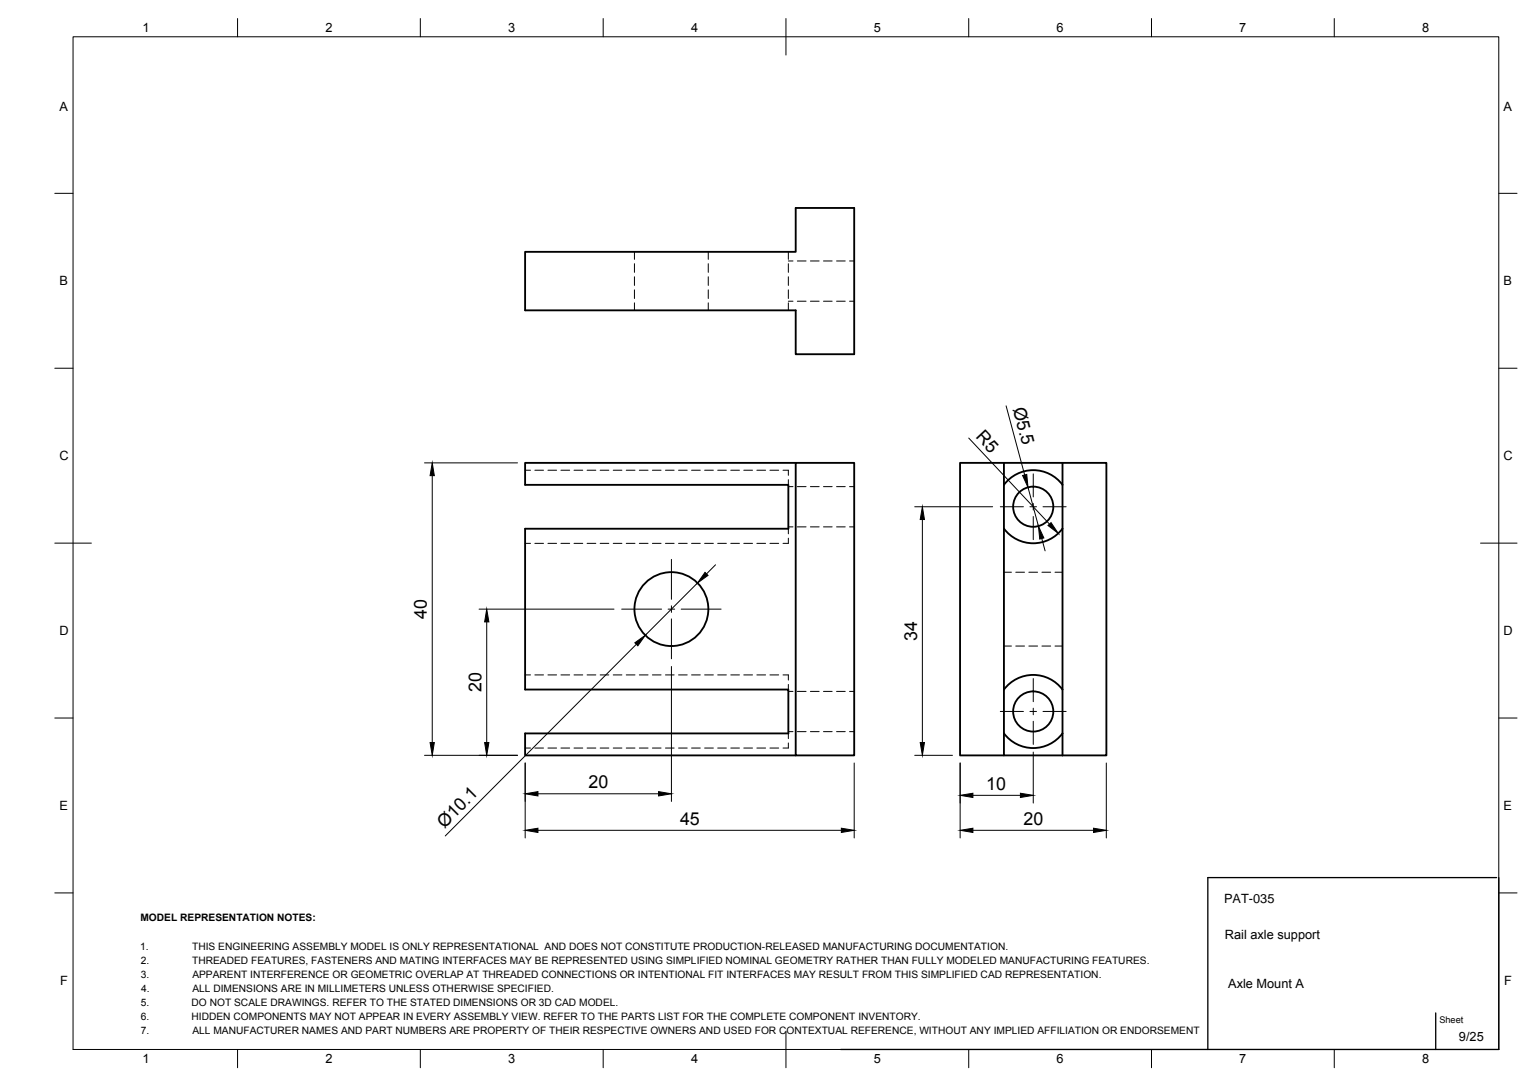
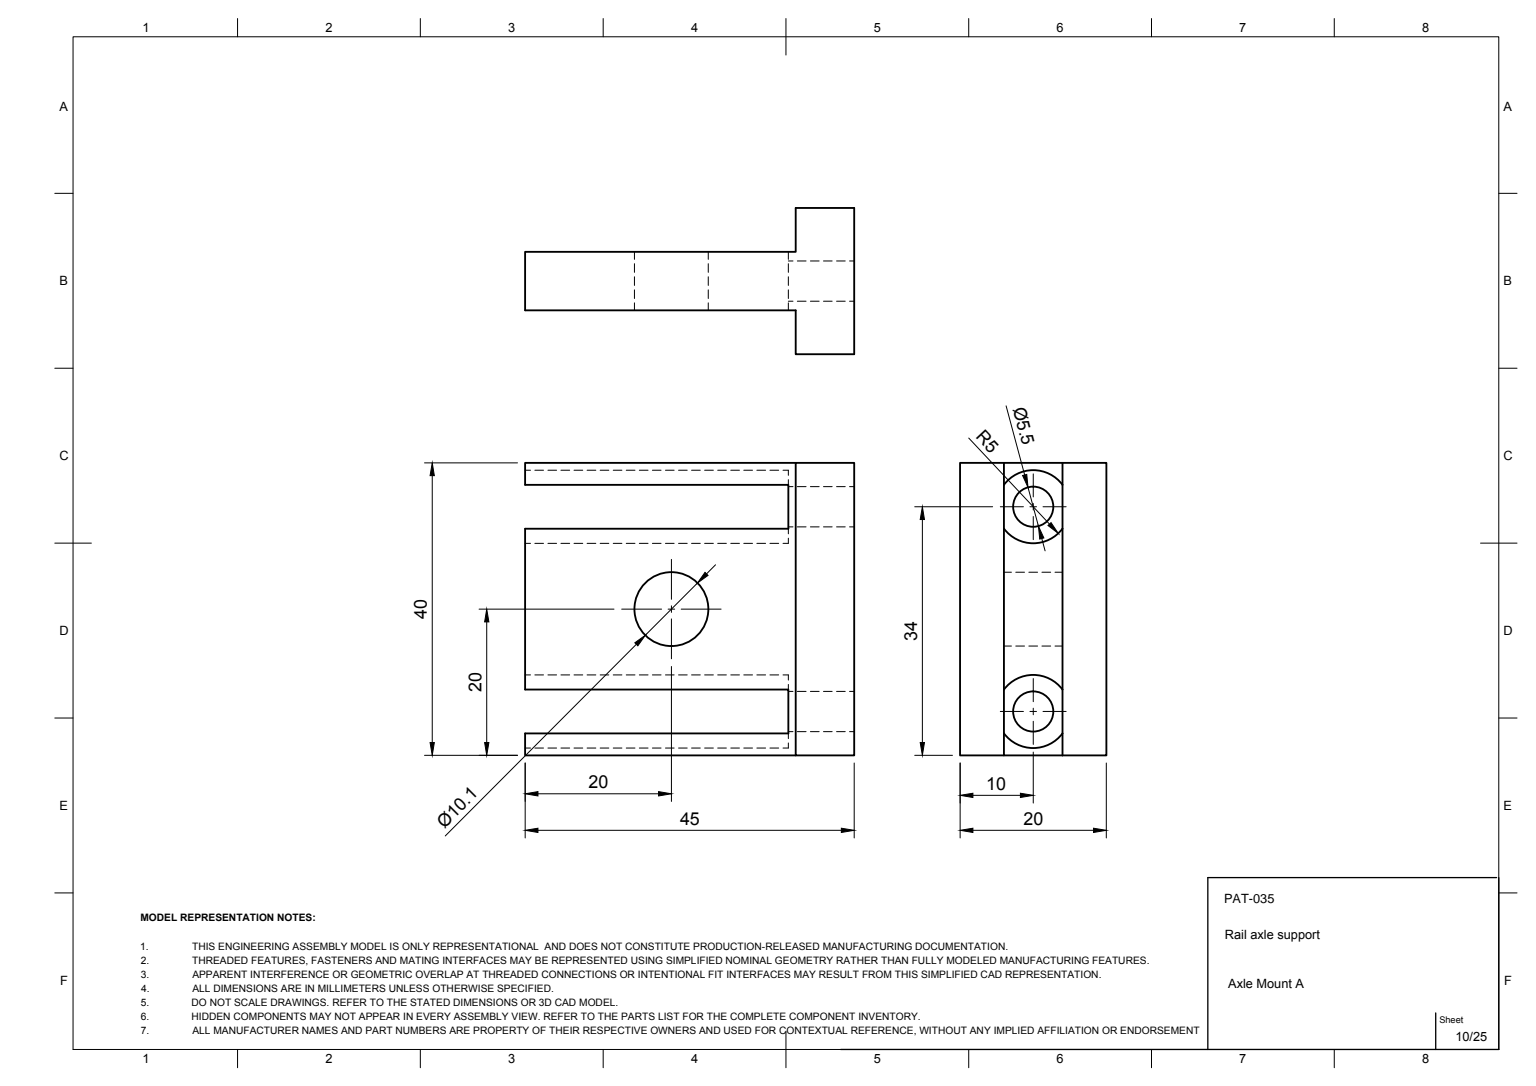
ISO-10303-21;
HEADER;
/* Generated by software containing ST-Developer
 * from STEP Tools, Inc. (www.steptools.com) 
 */

FILE_DESCRIPTION(
/* description */ ('Five-roller gravity conveyor'),
/* implementation_level */ '2;1');

FILE_NAME(
/* name */ 'Axle Mount A.step',
/* time_stamp */ '2026-10-29T15:36:43-07:00',
/* author */ (''),
/* organization */ (''),
/* preprocessor_version */ 'ST-DEVELOPER v20.2',
/* originating_system */ 'Autodesk Translation Framework v15.17.0.0',
/* authorisation */ '');

FILE_SCHEMA (('AUTOMOTIVE_DESIGN { 1 0 10303 214 3 1 1 }'));
ENDSEC;

DATA;
#10=MECHANICAL_DESIGN_GEOMETRIC_PRESENTATION_REPRESENTATION('',(#314),#7806);
#278=SHAPE_REPRESENTATION_RELATIONSHIP('SRR','None',#7915,#296);
#296=ADVANCED_BREP_SHAPE_REPRESENTATION('',(#340),#7788);
#314=STYLED_ITEM('',(#8091),#340);
#340=MANIFOLD_SOLID_BREP('Body1',#4201);
#368=FACE_BOUND('',#951,.T.);
#369=FACE_BOUND('',#955,.T.);
#370=FACE_BOUND('',#957,.T.);
#371=FACE_BOUND('',#969,.T.);
#372=FACE_BOUND('',#973,.T.);
#373=FACE_BOUND('',#974,.T.);
#433=CIRCLE('',#4503,0.5);
#434=CIRCLE('',#4504,0.5);
#435=CIRCLE('',#4506,0.5);
#436=CIRCLE('',#4507,0.5);
#437=CIRCLE('',#4509,0.275);
#438=CIRCLE('',#4511,0.5);
#439=CIRCLE('',#4512,0.5);
#440=CIRCLE('',#4514,0.5);
#441=CIRCLE('',#4515,0.5);
#442=CIRCLE('',#4517,0.275);
#443=CIRCLE('',#4519,0.505);
#444=CIRCLE('',#4524,0.275);
#445=CIRCLE('',#4526,0.275);
#446=CIRCLE('',#4528,0.505);
#600=CYLINDRICAL_SURFACE('',#4502,0.5);
#601=CYLINDRICAL_SURFACE('',#4505,0.5);
#602=CYLINDRICAL_SURFACE('',#4510,0.5);
#603=CYLINDRICAL_SURFACE('',#4513,0.5);
#604=CYLINDRICAL_SURFACE('',#4523,0.275);
#605=CYLINDRICAL_SURFACE('',#4525,0.275);
#606=CYLINDRICAL_SURFACE('',#4527,0.505);
#710=FACE_OUTER_BOUND('',#948,.T.);
#711=FACE_OUTER_BOUND('',#949,.T.);
#712=FACE_OUTER_BOUND('',#950,.T.);
#713=FACE_OUTER_BOUND('',#952,.T.);
#714=FACE_OUTER_BOUND('',#953,.T.);
#715=FACE_OUTER_BOUND('',#954,.T.);
#716=FACE_OUTER_BOUND('',#956,.T.);
#717=FACE_OUTER_BOUND('',#958,.T.);
#718=FACE_OUTER_BOUND('',#959,.T.);
#719=FACE_OUTER_BOUND('',#960,.T.);
#720=FACE_OUTER_BOUND('',#961,.T.);
#721=FACE_OUTER_BOUND('',#962,.T.);
#722=FACE_OUTER_BOUND('',#963,.T.);
#723=FACE_OUTER_BOUND('',#964,.T.);
#724=FACE_OUTER_BOUND('',#965,.T.);
#725=FACE_OUTER_BOUND('',#966,.T.);
#726=FACE_OUTER_BOUND('',#967,.T.);
#727=FACE_OUTER_BOUND('',#968,.T.);
#728=FACE_OUTER_BOUND('',#970,.T.);
#729=FACE_OUTER_BOUND('',#971,.T.);
#730=FACE_OUTER_BOUND('',#972,.T.);
#948=EDGE_LOOP('',(#3054,#3055,#3056,#3057));
#949=EDGE_LOOP('',(#3058,#3059,#3060,#3061));
#950=EDGE_LOOP('',(#3062,#3063,#3064,#3065));
#951=EDGE_LOOP('',(#3066));
#952=EDGE_LOOP('',(#3067,#3068,#3069,#3070));
#953=EDGE_LOOP('',(#3071,#3072,#3073,#3074));
#954=EDGE_LOOP('',(#3075,#3076,#3077,#3078));
#955=EDGE_LOOP('',(#3079));
#956=EDGE_LOOP('',(#3080,#3081,#3082,#3083,#3084,#3085,#3086,#3087,#3088,
#3089,#3090,#3091));
#957=EDGE_LOOP('',(#3092));
#958=EDGE_LOOP('',(#3093,#3094,#3095,#3096));
#959=EDGE_LOOP('',(#3097,#3098,#3099,#3100));
#960=EDGE_LOOP('',(#3101,#3102,#3103,#3104));
#961=EDGE_LOOP('',(#3105,#3106,#3107,#3108));
#962=EDGE_LOOP('',(#3109,#3110,#3111,#3112));
#963=EDGE_LOOP('',(#3113,#3114,#3115,#3116));
#964=EDGE_LOOP('',(#3117,#3118,#3119,#3120));
#965=EDGE_LOOP('',(#3121,#3122,#3123,#3124));
#966=EDGE_LOOP('',(#3125,#3126,#3127,#3128));
#967=EDGE_LOOP('',(#3129,#3130,#3131,#3132));
#968=EDGE_LOOP('',(#3133,#3134,#3135,#3136,#3137,#3138,#3139,#3140,#3141,
#3142,#3143,#3144));
#969=EDGE_LOOP('',(#3145));
#970=EDGE_LOOP('',(#3146,#3147,#3148,#3149,#3150,#3151,#3152,#3153));
#971=EDGE_LOOP('',(#3154,#3155,#3156,#3157,#3158,#3159,#3160,#3161));
#972=EDGE_LOOP('',(#3162,#3163,#3164,#3165));
#973=EDGE_LOOP('',(#3166));
#974=EDGE_LOOP('',(#3167));
#1313=LINE('',#6533,#1654);
#1314=LINE('',#6537,#1655);
#1315=LINE('',#6542,#1656);
#1316=LINE('',#6546,#1657);
#1317=LINE('',#6549,#1658);
#1318=LINE('',#6550,#1659);
#1319=LINE('',#6556,#1660);
#1320=LINE('',#6560,#1661);
#1321=LINE('',#6565,#1662);
#1322=LINE('',#6569,#1663);
#1323=LINE('',#6572,#1664);
#1324=LINE('',#6573,#1665);
#1325=LINE('',#6578,#1666);
#1326=LINE('',#6580,#1667);
#1327=LINE('',#6582,#1668);
#1328=LINE('',#6584,#1669);
#1329=LINE('',#6585,#1670);
#1330=LINE('',#6586,#1671);
#1331=LINE('',#6591,#1672);
#1332=LINE('',#6592,#1673);
#1333=LINE('',#6595,#1674);
#1334=LINE('',#6596,#1675);
#1335=LINE('',#6598,#1676);
#1336=LINE('',#6602,#1677);
#1337=LINE('',#6606,#1678);
#1338=LINE('',#6609,#1679);
#1339=LINE('',#6613,#1680);
#1340=LINE('',#6615,#1681);
#1341=LINE('',#6616,#1682);
#1342=LINE('',#6620,#1683);
#1343=LINE('',#6622,#1684);
#1344=LINE('',#6624,#1685);
#1345=LINE('',#6625,#1686);
#1346=LINE('',#6628,#1687);
#1347=LINE('',#6630,#1688);
#1348=LINE('',#6631,#1689);
#1349=LINE('',#6634,#1690);
#1350=LINE('',#6636,#1691);
#1351=LINE('',#6637,#1692);
#1352=LINE('',#6639,#1693);
#1353=LINE('',#6640,#1694);
#1354=LINE('',#6642,#1695);
#1355=LINE('',#6644,#1696);
#1654=VECTOR('',#5201,1.);
#1655=VECTOR('',#5204,1.);
#1656=VECTOR('',#5209,1.);
#1657=VECTOR('',#5212,1.);
#1658=VECTOR('',#5217,1.);
#1659=VECTOR('',#5218,1.);
#1660=VECTOR('',#5223,1.);
#1661=VECTOR('',#5226,1.);
#1662=VECTOR('',#5231,1.);
#1663=VECTOR('',#5234,1.);
#1664=VECTOR('',#5239,1.);
#1665=VECTOR('',#5240,1.);
#1666=VECTOR('',#5245,1.);
#1667=VECTOR('',#5246,1.);
#1668=VECTOR('',#5247,1.);
#1669=VECTOR('',#5248,1.);
#1670=VECTOR('',#5249,1.);
#1671=VECTOR('',#5250,1.);
#1672=VECTOR('',#5255,1.);
#1673=VECTOR('',#5256,1.);
#1674=VECTOR('',#5259,1.);
#1675=VECTOR('',#5260,1.);
#1676=VECTOR('',#5263,1.);
#1677=VECTOR('',#5268,0.275);
#1678=VECTOR('',#5273,0.275);
#1679=VECTOR('',#5276,0.505);
#1680=VECTOR('',#5281,1.);
#1681=VECTOR('',#5282,1.);
#1682=VECTOR('',#5283,1.);
#1683=VECTOR('',#5286,1.);
#1684=VECTOR('',#5287,1.);
#1685=VECTOR('',#5288,1.);
#1686=VECTOR('',#5289,1.);
#1687=VECTOR('',#5292,1.);
#1688=VECTOR('',#5293,1.);
#1689=VECTOR('',#5294,1.);
#1690=VECTOR('',#5297,1.);
#1691=VECTOR('',#5298,1.);
#1692=VECTOR('',#5299,1.);
#1693=VECTOR('',#5302,1.);
#1694=VECTOR('',#5303,1.);
#1695=VECTOR('',#5306,1.);
#1696=VECTOR('',#5309,1.);
#1957=VERTEX_POINT('',#6531);
#1958=VERTEX_POINT('',#6532);
#1959=VERTEX_POINT('',#6534);
#1960=VERTEX_POINT('',#6536);
#1961=VERTEX_POINT('',#6540);
#1962=VERTEX_POINT('',#6541);
#1963=VERTEX_POINT('',#6543);
#1964=VERTEX_POINT('',#6545);
#1965=VERTEX_POINT('',#6551);
#1966=VERTEX_POINT('',#6554);
#1967=VERTEX_POINT('',#6555);
#1968=VERTEX_POINT('',#6557);
#1969=VERTEX_POINT('',#6559);
#1970=VERTEX_POINT('',#6563);
#1971=VERTEX_POINT('',#6564);
#1972=VERTEX_POINT('',#6566);
#1973=VERTEX_POINT('',#6568);
#1974=VERTEX_POINT('',#6574);
#1975=VERTEX_POINT('',#6577);
#1976=VERTEX_POINT('',#6579);
#1977=VERTEX_POINT('',#6581);
#1978=VERTEX_POINT('',#6583);
#1979=VERTEX_POINT('',#6587);
#1980=VERTEX_POINT('',#6590);
#1981=VERTEX_POINT('',#6594);
#1982=VERTEX_POINT('',#6600);
#1983=VERTEX_POINT('',#6604);
#1984=VERTEX_POINT('',#6608);
#1985=VERTEX_POINT('',#6612);
#1986=VERTEX_POINT('',#6614);
#1987=VERTEX_POINT('',#6618);
#1988=VERTEX_POINT('',#6619);
#1989=VERTEX_POINT('',#6621);
#1990=VERTEX_POINT('',#6623);
#1991=VERTEX_POINT('',#6627);
#1992=VERTEX_POINT('',#6629);
#1993=VERTEX_POINT('',#6633);
#1994=VERTEX_POINT('',#6635);
#2370=EDGE_CURVE('',#1957,#1958,#1313,.T.);
#2371=EDGE_CURVE('',#1959,#1957,#433,.T.);
#2372=EDGE_CURVE('',#1960,#1959,#1314,.T.);
#2373=EDGE_CURVE('',#1958,#1960,#434,.T.);
#2374=EDGE_CURVE('',#1961,#1962,#1315,.T.);
#2375=EDGE_CURVE('',#1963,#1961,#435,.T.);
#2376=EDGE_CURVE('',#1964,#1963,#1316,.T.);
#2377=EDGE_CURVE('',#1962,#1964,#436,.T.);
#2378=EDGE_CURVE('',#1958,#1961,#1317,.T.);
#2379=EDGE_CURVE('',#1963,#1960,#1318,.T.);
#2380=EDGE_CURVE('',#1965,#1965,#437,.T.);
#2381=EDGE_CURVE('',#1966,#1967,#1319,.T.);
#2382=EDGE_CURVE('',#1968,#1966,#438,.T.);
#2383=EDGE_CURVE('',#1969,#1968,#1320,.T.);
#2384=EDGE_CURVE('',#1967,#1969,#439,.T.);
#2385=EDGE_CURVE('',#1970,#1971,#1321,.T.);
#2386=EDGE_CURVE('',#1972,#1970,#440,.T.);
#2387=EDGE_CURVE('',#1973,#1972,#1322,.T.);
#2388=EDGE_CURVE('',#1971,#1973,#441,.T.);
#2389=EDGE_CURVE('',#1967,#1970,#1323,.T.);
#2390=EDGE_CURVE('',#1972,#1969,#1324,.T.);
#2391=EDGE_CURVE('',#1974,#1974,#442,.T.);
#2392=EDGE_CURVE('',#1975,#1959,#1325,.T.);
#2393=EDGE_CURVE('',#1976,#1975,#1326,.T.);
#2394=EDGE_CURVE('',#1976,#1977,#1327,.T.);
#2395=EDGE_CURVE('',#1977,#1978,#1328,.T.);
#2396=EDGE_CURVE('',#1973,#1978,#1329,.T.);
#2397=EDGE_CURVE('',#1964,#1968,#1330,.T.);
#2398=EDGE_CURVE('',#1979,#1979,#443,.T.);
#2399=EDGE_CURVE('',#1978,#1980,#1331,.T.);
#2400=EDGE_CURVE('',#1980,#1971,#1332,.T.);
#2401=EDGE_CURVE('',#1957,#1981,#1333,.T.);
#2402=EDGE_CURVE('',#1981,#1975,#1334,.T.);
#2403=EDGE_CURVE('',#1966,#1962,#1335,.T.);
#2404=EDGE_CURVE('',#1982,#1982,#444,.T.);
#2405=EDGE_CURVE('',#1982,#1965,#1336,.T.);
#2406=EDGE_CURVE('',#1983,#1983,#445,.T.);
#2407=EDGE_CURVE('',#1983,#1974,#1337,.T.);
#2408=EDGE_CURVE('',#1979,#1984,#1338,.T.);
#2409=EDGE_CURVE('',#1984,#1984,#446,.T.);
#2410=EDGE_CURVE('',#1985,#1976,#1339,.T.);
#2411=EDGE_CURVE('',#1986,#1985,#1340,.T.);
#2412=EDGE_CURVE('',#1986,#1977,#1341,.T.);
#2413=EDGE_CURVE('',#1987,#1988,#1342,.T.);
#2414=EDGE_CURVE('',#1987,#1989,#1343,.T.);
#2415=EDGE_CURVE('',#1990,#1989,#1344,.T.);
#2416=EDGE_CURVE('',#1988,#1990,#1345,.T.);
#2417=EDGE_CURVE('',#1989,#1991,#1346,.T.);
#2418=EDGE_CURVE('',#1991,#1992,#1347,.T.);
#2419=EDGE_CURVE('',#1992,#1990,#1348,.T.);
#2420=EDGE_CURVE('',#1985,#1993,#1349,.T.);
#2421=EDGE_CURVE('',#1993,#1994,#1350,.T.);
#2422=EDGE_CURVE('',#1994,#1986,#1351,.T.);
#2423=EDGE_CURVE('',#1987,#1980,#1352,.T.);
#2424=EDGE_CURVE('',#1988,#1981,#1353,.T.);
#2425=EDGE_CURVE('',#1992,#1993,#1354,.T.);
#2426=EDGE_CURVE('',#1994,#1991,#1355,.T.);
#3054=ORIENTED_EDGE('',*,*,#2370,.F.);
#3055=ORIENTED_EDGE('',*,*,#2371,.F.);
#3056=ORIENTED_EDGE('',*,*,#2372,.F.);
#3057=ORIENTED_EDGE('',*,*,#2373,.F.);
#3058=ORIENTED_EDGE('',*,*,#2374,.F.);
#3059=ORIENTED_EDGE('',*,*,#2375,.F.);
#3060=ORIENTED_EDGE('',*,*,#2376,.F.);
#3061=ORIENTED_EDGE('',*,*,#2377,.F.);
#3062=ORIENTED_EDGE('',*,*,#2378,.F.);
#3063=ORIENTED_EDGE('',*,*,#2373,.T.);
#3064=ORIENTED_EDGE('',*,*,#2379,.F.);
#3065=ORIENTED_EDGE('',*,*,#2375,.T.);
#3066=ORIENTED_EDGE('',*,*,#2380,.F.);
#3067=ORIENTED_EDGE('',*,*,#2381,.F.);
#3068=ORIENTED_EDGE('',*,*,#2382,.F.);
#3069=ORIENTED_EDGE('',*,*,#2383,.F.);
#3070=ORIENTED_EDGE('',*,*,#2384,.F.);
#3071=ORIENTED_EDGE('',*,*,#2385,.F.);
#3072=ORIENTED_EDGE('',*,*,#2386,.F.);
#3073=ORIENTED_EDGE('',*,*,#2387,.F.);
#3074=ORIENTED_EDGE('',*,*,#2388,.F.);
#3075=ORIENTED_EDGE('',*,*,#2389,.F.);
#3076=ORIENTED_EDGE('',*,*,#2384,.T.);
#3077=ORIENTED_EDGE('',*,*,#2390,.F.);
#3078=ORIENTED_EDGE('',*,*,#2386,.T.);
#3079=ORIENTED_EDGE('',*,*,#2391,.F.);
#3080=ORIENTED_EDGE('',*,*,#2376,.T.);
#3081=ORIENTED_EDGE('',*,*,#2379,.T.);
#3082=ORIENTED_EDGE('',*,*,#2372,.T.);
#3083=ORIENTED_EDGE('',*,*,#2392,.F.);
#3084=ORIENTED_EDGE('',*,*,#2393,.F.);
#3085=ORIENTED_EDGE('',*,*,#2394,.T.);
#3086=ORIENTED_EDGE('',*,*,#2395,.T.);
#3087=ORIENTED_EDGE('',*,*,#2396,.F.);
#3088=ORIENTED_EDGE('',*,*,#2387,.T.);
#3089=ORIENTED_EDGE('',*,*,#2390,.T.);
#3090=ORIENTED_EDGE('',*,*,#2383,.T.);
#3091=ORIENTED_EDGE('',*,*,#2397,.F.);
#3092=ORIENTED_EDGE('',*,*,#2398,.T.);
#3093=ORIENTED_EDGE('',*,*,#2388,.T.);
#3094=ORIENTED_EDGE('',*,*,#2396,.T.);
#3095=ORIENTED_EDGE('',*,*,#2399,.T.);
#3096=ORIENTED_EDGE('',*,*,#2400,.T.);
#3097=ORIENTED_EDGE('',*,*,#2371,.T.);
#3098=ORIENTED_EDGE('',*,*,#2401,.T.);
#3099=ORIENTED_EDGE('',*,*,#2402,.T.);
#3100=ORIENTED_EDGE('',*,*,#2392,.T.);
#3101=ORIENTED_EDGE('',*,*,#2377,.T.);
#3102=ORIENTED_EDGE('',*,*,#2397,.T.);
#3103=ORIENTED_EDGE('',*,*,#2382,.T.);
#3104=ORIENTED_EDGE('',*,*,#2403,.T.);
#3105=ORIENTED_EDGE('',*,*,#2404,.F.);
#3106=ORIENTED_EDGE('',*,*,#2405,.T.);
#3107=ORIENTED_EDGE('',*,*,#2380,.T.);
#3108=ORIENTED_EDGE('',*,*,#2405,.F.);
#3109=ORIENTED_EDGE('',*,*,#2406,.F.);
#3110=ORIENTED_EDGE('',*,*,#2407,.T.);
#3111=ORIENTED_EDGE('',*,*,#2391,.T.);
#3112=ORIENTED_EDGE('',*,*,#2407,.F.);
#3113=ORIENTED_EDGE('',*,*,#2398,.F.);
#3114=ORIENTED_EDGE('',*,*,#2408,.T.);
#3115=ORIENTED_EDGE('',*,*,#2409,.F.);
#3116=ORIENTED_EDGE('',*,*,#2408,.F.);
#3117=ORIENTED_EDGE('',*,*,#2394,.F.);
#3118=ORIENTED_EDGE('',*,*,#2410,.F.);
#3119=ORIENTED_EDGE('',*,*,#2411,.F.);
#3120=ORIENTED_EDGE('',*,*,#2412,.T.);
#3121=ORIENTED_EDGE('',*,*,#2413,.F.);
#3122=ORIENTED_EDGE('',*,*,#2414,.T.);
#3123=ORIENTED_EDGE('',*,*,#2415,.F.);
#3124=ORIENTED_EDGE('',*,*,#2416,.F.);
#3125=ORIENTED_EDGE('',*,*,#2415,.T.);
#3126=ORIENTED_EDGE('',*,*,#2417,.T.);
#3127=ORIENTED_EDGE('',*,*,#2418,.T.);
#3128=ORIENTED_EDGE('',*,*,#2419,.T.);
#3129=ORIENTED_EDGE('',*,*,#2411,.T.);
#3130=ORIENTED_EDGE('',*,*,#2420,.T.);
#3131=ORIENTED_EDGE('',*,*,#2421,.T.);
#3132=ORIENTED_EDGE('',*,*,#2422,.T.);
#3133=ORIENTED_EDGE('',*,*,#2374,.T.);
#3134=ORIENTED_EDGE('',*,*,#2403,.F.);
#3135=ORIENTED_EDGE('',*,*,#2381,.T.);
#3136=ORIENTED_EDGE('',*,*,#2389,.T.);
#3137=ORIENTED_EDGE('',*,*,#2385,.T.);
#3138=ORIENTED_EDGE('',*,*,#2400,.F.);
#3139=ORIENTED_EDGE('',*,*,#2423,.F.);
#3140=ORIENTED_EDGE('',*,*,#2413,.T.);
#3141=ORIENTED_EDGE('',*,*,#2424,.T.);
#3142=ORIENTED_EDGE('',*,*,#2401,.F.);
#3143=ORIENTED_EDGE('',*,*,#2370,.T.);
#3144=ORIENTED_EDGE('',*,*,#2378,.T.);
#3145=ORIENTED_EDGE('',*,*,#2409,.T.);
#3146=ORIENTED_EDGE('',*,*,#2393,.T.);
#3147=ORIENTED_EDGE('',*,*,#2402,.F.);
#3148=ORIENTED_EDGE('',*,*,#2424,.F.);
#3149=ORIENTED_EDGE('',*,*,#2416,.T.);
#3150=ORIENTED_EDGE('',*,*,#2419,.F.);
#3151=ORIENTED_EDGE('',*,*,#2425,.T.);
#3152=ORIENTED_EDGE('',*,*,#2420,.F.);
#3153=ORIENTED_EDGE('',*,*,#2410,.T.);
#3154=ORIENTED_EDGE('',*,*,#2423,.T.);
#3155=ORIENTED_EDGE('',*,*,#2399,.F.);
#3156=ORIENTED_EDGE('',*,*,#2395,.F.);
#3157=ORIENTED_EDGE('',*,*,#2412,.F.);
#3158=ORIENTED_EDGE('',*,*,#2422,.F.);
#3159=ORIENTED_EDGE('',*,*,#2426,.T.);
#3160=ORIENTED_EDGE('',*,*,#2417,.F.);
#3161=ORIENTED_EDGE('',*,*,#2414,.F.);
#3162=ORIENTED_EDGE('',*,*,#2425,.F.);
#3163=ORIENTED_EDGE('',*,*,#2418,.F.);
#3164=ORIENTED_EDGE('',*,*,#2426,.F.);
#3165=ORIENTED_EDGE('',*,*,#2421,.F.);
#3166=ORIENTED_EDGE('',*,*,#2404,.T.);
#3167=ORIENTED_EDGE('',*,*,#2406,.T.);
#3874=PLANE('',#4508);
#3875=PLANE('',#4516);
#3876=PLANE('',#4518);
#3877=PLANE('',#4520);
#3878=PLANE('',#4521);
#3879=PLANE('',#4522);
#3880=PLANE('',#4529);
#3881=PLANE('',#4530);
#3882=PLANE('',#4531);
#3883=PLANE('',#4532);
#3884=PLANE('',#4533);
#3885=PLANE('',#4534);
#3886=PLANE('',#4535);
#3887=PLANE('',#4536);
#4025=ADVANCED_FACE('',(#710),#600,.F.);
#4026=ADVANCED_FACE('',(#711),#601,.F.);
#4027=ADVANCED_FACE('',(#712,#368),#3874,.T.);
#4028=ADVANCED_FACE('',(#713),#602,.F.);
#4029=ADVANCED_FACE('',(#714),#603,.F.);
#4030=ADVANCED_FACE('',(#715,#369),#3875,.T.);
#4031=ADVANCED_FACE('',(#716,#370),#3876,.T.);
#4032=ADVANCED_FACE('',(#717),#3877,.T.);
#4033=ADVANCED_FACE('',(#718),#3878,.T.);
#4034=ADVANCED_FACE('',(#719),#3879,.T.);
#4035=ADVANCED_FACE('',(#720),#604,.F.);
#4036=ADVANCED_FACE('',(#721),#605,.F.);
#4037=ADVANCED_FACE('',(#722),#606,.F.);
#4038=ADVANCED_FACE('',(#723),#3880,.T.);
#4039=ADVANCED_FACE('',(#724),#3881,.T.);
#4040=ADVANCED_FACE('',(#725),#3882,.T.);
#4041=ADVANCED_FACE('',(#726),#3883,.F.);
#4042=ADVANCED_FACE('',(#727,#371),#3884,.T.);
#4043=ADVANCED_FACE('',(#728),#3885,.T.);
#4044=ADVANCED_FACE('',(#729),#3886,.T.);
#4045=ADVANCED_FACE('',(#730,#372,#373),#3887,.F.);
#4201=CLOSED_SHELL('',(#4025,#4026,#4027,#4028,#4029,#4030,#4031,#4032,
#4033,#4034,#4035,#4036,#4037,#4038,#4039,#4040,#4041,#4042,#4043,#4044,
#4045));
#4501=AXIS2_PLACEMENT_3D('',#6529,#5197,#5198);
#4502=AXIS2_PLACEMENT_3D('',#6530,#5199,#5200);
#4503=AXIS2_PLACEMENT_3D('',#6535,#5202,#5203);
#4504=AXIS2_PLACEMENT_3D('',#6538,#5205,#5206);
#4505=AXIS2_PLACEMENT_3D('',#6539,#5207,#5208);
#4506=AXIS2_PLACEMENT_3D('',#6544,#5210,#5211);
#4507=AXIS2_PLACEMENT_3D('',#6547,#5213,#5214);
#4508=AXIS2_PLACEMENT_3D('',#6548,#5215,#5216);
#4509=AXIS2_PLACEMENT_3D('',#6552,#5219,#5220);
#4510=AXIS2_PLACEMENT_3D('',#6553,#5221,#5222);
#4511=AXIS2_PLACEMENT_3D('',#6558,#5224,#5225);
#4512=AXIS2_PLACEMENT_3D('',#6561,#5227,#5228);
#4513=AXIS2_PLACEMENT_3D('',#6562,#5229,#5230);
#4514=AXIS2_PLACEMENT_3D('',#6567,#5232,#5233);
#4515=AXIS2_PLACEMENT_3D('',#6570,#5235,#5236);
#4516=AXIS2_PLACEMENT_3D('',#6571,#5237,#5238);
#4517=AXIS2_PLACEMENT_3D('',#6575,#5241,#5242);
#4518=AXIS2_PLACEMENT_3D('',#6576,#5243,#5244);
#4519=AXIS2_PLACEMENT_3D('',#6588,#5251,#5252);
#4520=AXIS2_PLACEMENT_3D('',#6589,#5253,#5254);
#4521=AXIS2_PLACEMENT_3D('',#6593,#5257,#5258);
#4522=AXIS2_PLACEMENT_3D('',#6597,#5261,#5262);
#4523=AXIS2_PLACEMENT_3D('',#6599,#5264,#5265);
#4524=AXIS2_PLACEMENT_3D('',#6601,#5266,#5267);
#4525=AXIS2_PLACEMENT_3D('',#6603,#5269,#5270);
#4526=AXIS2_PLACEMENT_3D('',#6605,#5271,#5272);
#4527=AXIS2_PLACEMENT_3D('',#6607,#5274,#5275);
#4528=AXIS2_PLACEMENT_3D('',#6610,#5277,#5278);
#4529=AXIS2_PLACEMENT_3D('',#6611,#5279,#5280);
#4530=AXIS2_PLACEMENT_3D('',#6617,#5284,#5285);
#4531=AXIS2_PLACEMENT_3D('',#6626,#5290,#5291);
#4532=AXIS2_PLACEMENT_3D('',#6632,#5295,#5296);
#4533=AXIS2_PLACEMENT_3D('',#6638,#5300,#5301);
#4534=AXIS2_PLACEMENT_3D('',#6641,#5304,#5305);
#4535=AXIS2_PLACEMENT_3D('',#6643,#5307,#5308);
#4536=AXIS2_PLACEMENT_3D('',#6645,#5310,#5311);
#5197=DIRECTION('axis',(0.,0.,1.));
#5198=DIRECTION('refdir',(1.,0.,0.));
#5199=DIRECTION('center_axis',(0.,0.,1.));
#5200=DIRECTION('ref_axis',(-1.,1.22464679914735E-16,0.));
#5201=DIRECTION('',(0.,0.,-1.));
#5202=DIRECTION('center_axis',(0.,0.,-1.));
#5203=DIRECTION('ref_axis',(1.,0.,0.));
#5204=DIRECTION('',(0.,0.,1.));
#5205=DIRECTION('center_axis',(0.,0.,1.));
#5206=DIRECTION('ref_axis',(1.,0.,0.));
#5207=DIRECTION('center_axis',(0.,0.,1.));
#5208=DIRECTION('ref_axis',(1.,0.,0.));
#5209=DIRECTION('',(0.,0.,1.));
#5210=DIRECTION('center_axis',(0.,0.,1.));
#5211=DIRECTION('ref_axis',(1.,0.,0.));
#5212=DIRECTION('',(0.,0.,-1.));
#5213=DIRECTION('center_axis',(0.,0.,-1.));
#5214=DIRECTION('ref_axis',(1.,0.,0.));
#5215=DIRECTION('center_axis',(0.,0.,1.));
#5216=DIRECTION('ref_axis',(1.,0.,0.));
#5217=DIRECTION('',(1.,0.,0.));
#5218=DIRECTION('',(-1.,0.,0.));
#5219=DIRECTION('center_axis',(0.,0.,1.));
#5220=DIRECTION('ref_axis',(1.,0.,0.));
#5221=DIRECTION('center_axis',(0.,0.,1.));
#5222=DIRECTION('ref_axis',(-1.,1.22464679914735E-16,0.));
#5223=DIRECTION('',(0.,0.,-1.));
#5224=DIRECTION('center_axis',(0.,0.,-1.));
#5225=DIRECTION('ref_axis',(1.,0.,0.));
#5226=DIRECTION('',(0.,0.,1.));
#5227=DIRECTION('center_axis',(0.,0.,1.));
#5228=DIRECTION('ref_axis',(1.,0.,0.));
#5229=DIRECTION('center_axis',(0.,0.,1.));
#5230=DIRECTION('ref_axis',(1.,0.,0.));
#5231=DIRECTION('',(0.,0.,1.));
#5232=DIRECTION('center_axis',(0.,0.,1.));
#5233=DIRECTION('ref_axis',(1.,0.,0.));
#5234=DIRECTION('',(0.,0.,-1.));
#5235=DIRECTION('center_axis',(0.,0.,-1.));
#5236=DIRECTION('ref_axis',(1.,0.,0.));
#5237=DIRECTION('center_axis',(0.,0.,1.));
#5238=DIRECTION('ref_axis',(1.,0.,0.));
#5239=DIRECTION('',(1.,0.,0.));
#5240=DIRECTION('',(-1.,0.,0.));
#5241=DIRECTION('center_axis',(0.,0.,1.));
#5242=DIRECTION('ref_axis',(1.,0.,0.));
#5243=DIRECTION('center_axis',(0.,-1.,0.));
#5244=DIRECTION('ref_axis',(1.,0.,0.));
#5245=DIRECTION('',(1.,0.,0.));
#5246=DIRECTION('',(0.,0.,1.));
#5247=DIRECTION('',(1.,0.,0.));
#5248=DIRECTION('',(0.,0.,1.));
#5249=DIRECTION('',(1.,0.,0.));
#5250=DIRECTION('',(1.,0.,0.));
#5251=DIRECTION('center_axis',(0.,1.,0.));
#5252=DIRECTION('ref_axis',(1.,0.,0.));
#5253=DIRECTION('center_axis',(0.,0.,1.));
#5254=DIRECTION('ref_axis',(1.,0.,0.));
#5255=DIRECTION('',(0.,1.,0.));
#5256=DIRECTION('',(-1.,0.,0.));
#5257=DIRECTION('center_axis',(0.,0.,1.));
#5258=DIRECTION('ref_axis',(1.,0.,0.));
#5259=DIRECTION('',(-1.,0.,0.));
#5260=DIRECTION('',(0.,-1.,0.));
#5261=DIRECTION('center_axis',(0.,0.,1.));
#5262=DIRECTION('ref_axis',(1.,0.,0.));
#5263=DIRECTION('',(-1.,0.,0.));
#5264=DIRECTION('center_axis',(0.,0.,1.));
#5265=DIRECTION('ref_axis',(1.,0.,0.));
#5266=DIRECTION('center_axis',(0.,0.,1.));
#5267=DIRECTION('ref_axis',(1.,0.,0.));
#5268=DIRECTION('',(0.,0.,1.));
#5269=DIRECTION('center_axis',(0.,0.,1.));
#5270=DIRECTION('ref_axis',(1.,0.,0.));
#5271=DIRECTION('center_axis',(0.,0.,1.));
#5272=DIRECTION('ref_axis',(1.,0.,0.));
#5273=DIRECTION('',(0.,0.,1.));
#5274=DIRECTION('center_axis',(0.,1.,0.));
#5275=DIRECTION('ref_axis',(1.,0.,0.));
#5276=DIRECTION('',(0.,1.,0.));
#5277=DIRECTION('center_axis',(0.,-1.,0.));
#5278=DIRECTION('ref_axis',(1.,0.,0.));
#5279=DIRECTION('center_axis',(0.,0.,1.));
#5280=DIRECTION('ref_axis',(1.,0.,0.));
#5281=DIRECTION('',(0.,1.,0.));
#5282=DIRECTION('',(-1.,0.,0.));
#5283=DIRECTION('',(0.,1.,0.));
#5284=DIRECTION('center_axis',(0.,0.,1.));
#5285=DIRECTION('ref_axis',(1.,0.,0.));
#5286=DIRECTION('',(-1.,0.,0.));
#5287=DIRECTION('',(0.,1.,0.));
#5288=DIRECTION('',(1.,0.,0.));
#5289=DIRECTION('',(0.,1.,0.));
#5290=DIRECTION('center_axis',(0.,1.,0.));
#5291=DIRECTION('ref_axis',(0.,0.,1.));
#5292=DIRECTION('',(0.,0.,-1.));
#5293=DIRECTION('',(-1.,0.,0.));
#5294=DIRECTION('',(0.,0.,1.));
#5295=DIRECTION('center_axis',(0.,1.,0.));
#5296=DIRECTION('ref_axis',(1.,0.,0.));
#5297=DIRECTION('',(0.,0.,-1.));
#5298=DIRECTION('',(1.,0.,0.));
#5299=DIRECTION('',(0.,0.,1.));
#5300=DIRECTION('center_axis',(0.,1.,0.));
#5301=DIRECTION('ref_axis',(-1.,0.,0.));
#5302=DIRECTION('',(0.,0.,1.));
#5303=DIRECTION('',(0.,0.,1.));
#5304=DIRECTION('center_axis',(-1.,0.,0.));
#5305=DIRECTION('ref_axis',(0.,-1.,0.));
#5306=DIRECTION('',(0.,-1.,0.));
#5307=DIRECTION('center_axis',(1.,0.,0.));
#5308=DIRECTION('ref_axis',(0.,1.,0.));
#5309=DIRECTION('',(0.,1.,0.));
#5310=DIRECTION('center_axis',(0.,0.,1.));
#5311=DIRECTION('ref_axis',(1.,0.,0.));
#6529=CARTESIAN_POINT('',(0.,0.,0.));
#6530=CARTESIAN_POINT('Origin',(1.6,-2.,2.9));
#6531=CARTESIAN_POINT('',(1.3,-1.6,6.5));
#6532=CARTESIAN_POINT('',(1.3,-1.6,2.9));
#6533=CARTESIAN_POINT('',(1.3,-1.6,2.9));
#6534=CARTESIAN_POINT('',(1.3,-2.4,6.5));
#6535=CARTESIAN_POINT('Origin',(1.6,-2.,6.5));
#6536=CARTESIAN_POINT('',(1.3,-2.4,2.9));
#6537=CARTESIAN_POINT('',(1.3,-2.4,2.9));
#6538=CARTESIAN_POINT('Origin',(1.6,-2.,2.9));
#6539=CARTESIAN_POINT('Origin',(1.6,-2.,2.9));
#6540=CARTESIAN_POINT('',(1.9,-1.6,2.9));
#6541=CARTESIAN_POINT('',(1.9,-1.6,6.5));
#6542=CARTESIAN_POINT('',(1.9,-1.6,2.9));
#6543=CARTESIAN_POINT('',(1.9,-2.4,2.9));
#6544=CARTESIAN_POINT('Origin',(1.6,-2.,2.9));
#6545=CARTESIAN_POINT('',(1.9,-2.4,6.5));
#6546=CARTESIAN_POINT('',(1.9,-2.4,2.9));
#6547=CARTESIAN_POINT('Origin',(1.6,-2.,6.5));
#6548=CARTESIAN_POINT('Origin',(1.6,-2.,2.9));
#6549=CARTESIAN_POINT('',(3.3,-1.6,2.9));
#6550=CARTESIAN_POINT('',(1.3,-2.4,2.9));
#6551=CARTESIAN_POINT('',(1.325,-2.,2.9));
#6552=CARTESIAN_POINT('Origin',(1.6,-2.,2.9));
#6553=CARTESIAN_POINT('Origin',(4.4,-2.,2.9));
#6554=CARTESIAN_POINT('',(4.1,-1.6,6.5));
#6555=CARTESIAN_POINT('',(4.1,-1.6,2.9));
#6556=CARTESIAN_POINT('',(4.1,-1.6,2.9));
#6557=CARTESIAN_POINT('',(4.1,-2.4,6.5));
#6558=CARTESIAN_POINT('Origin',(4.4,-2.,6.5));
#6559=CARTESIAN_POINT('',(4.1,-2.4,2.9));
#6560=CARTESIAN_POINT('',(4.1,-2.4,2.9));
#6561=CARTESIAN_POINT('Origin',(4.4,-2.,2.9));
#6562=CARTESIAN_POINT('Origin',(4.4,-2.,2.9));
#6563=CARTESIAN_POINT('',(4.7,-1.6,2.9));
#6564=CARTESIAN_POINT('',(4.7,-1.6,6.5));
#6565=CARTESIAN_POINT('',(4.7,-1.6,2.9));
#6566=CARTESIAN_POINT('',(4.7,-2.4,2.9));
#6567=CARTESIAN_POINT('Origin',(4.4,-2.,2.9));
#6568=CARTESIAN_POINT('',(4.7,-2.4,6.5));
#6569=CARTESIAN_POINT('',(4.7,-2.4,2.9));
#6570=CARTESIAN_POINT('Origin',(4.4,-2.,6.5));
#6571=CARTESIAN_POINT('Origin',(4.4,-2.,2.9));
#6572=CARTESIAN_POINT('',(4.7,-1.6,2.9));
#6573=CARTESIAN_POINT('',(2.7,-2.4,2.9));
#6574=CARTESIAN_POINT('',(4.125,-2.,2.9));
#6575=CARTESIAN_POINT('Origin',(4.4,-2.,2.9));
#6576=CARTESIAN_POINT('Origin',(1.,-2.4,2.));
#6577=CARTESIAN_POINT('',(1.,-2.4,6.5));
#6578=CARTESIAN_POINT('',(1.,-2.4,6.5));
#6579=CARTESIAN_POINT('',(1.,-2.4,2.8));
#6580=CARTESIAN_POINT('',(1.,-2.4,2.));
#6581=CARTESIAN_POINT('',(5.,-2.4,2.8));
#6582=CARTESIAN_POINT('',(1.,-2.4,2.8));
#6583=CARTESIAN_POINT('',(5.,-2.4,6.5));
#6584=CARTESIAN_POINT('',(5.,-2.4,2.));
#6585=CARTESIAN_POINT('',(1.,-2.4,6.5));
#6586=CARTESIAN_POINT('',(1.,-2.4,6.5));
#6587=CARTESIAN_POINT('',(2.495,-2.4,4.5));
#6588=CARTESIAN_POINT('Origin',(3.,-2.4,4.5));
#6589=CARTESIAN_POINT('Origin',(3.,-2.,6.5));
#6590=CARTESIAN_POINT('',(5.,-1.6,6.5));
#6591=CARTESIAN_POINT('',(5.,-2.4,6.5));
#6592=CARTESIAN_POINT('',(5.,-1.6,6.5));
#6593=CARTESIAN_POINT('Origin',(3.,-2.,6.5));
#6594=CARTESIAN_POINT('',(1.,-1.6,6.5));
#6595=CARTESIAN_POINT('',(5.,-1.6,6.5));
#6596=CARTESIAN_POINT('',(1.,-1.6,6.5));
#6597=CARTESIAN_POINT('Origin',(3.,-2.,6.5));
#6598=CARTESIAN_POINT('',(5.,-1.6,6.5));
#6599=CARTESIAN_POINT('Origin',(1.6,-2.,1.9));
#6600=CARTESIAN_POINT('',(1.325,-2.,2.));
#6601=CARTESIAN_POINT('Origin',(1.6,-2.,2.));
#6602=CARTESIAN_POINT('',(1.325,-2.,1.9));
#6603=CARTESIAN_POINT('Origin',(4.4,-2.,1.9));
#6604=CARTESIAN_POINT('',(4.125,-2.,2.));
#6605=CARTESIAN_POINT('Origin',(4.4,-2.,2.));
#6606=CARTESIAN_POINT('',(4.125,-2.,1.9));
#6607=CARTESIAN_POINT('Origin',(3.,-2.5,4.5));
#6608=CARTESIAN_POINT('',(2.495,-1.6,4.5));
#6609=CARTESIAN_POINT('',(2.495,-2.5,4.5));
#6610=CARTESIAN_POINT('Origin',(3.,-1.6,4.5));
#6611=CARTESIAN_POINT('Origin',(1.,-3.,2.8));
#6612=CARTESIAN_POINT('',(1.,-3.,2.8));
#6613=CARTESIAN_POINT('',(1.,-3.,2.8));
#6614=CARTESIAN_POINT('',(5.,-3.,2.8));
#6615=CARTESIAN_POINT('',(5.,-3.,2.8));
#6616=CARTESIAN_POINT('',(5.,-3.,2.8));
#6617=CARTESIAN_POINT('Origin',(1.,-3.,2.8));
#6618=CARTESIAN_POINT('',(5.,-1.6,2.8));
#6619=CARTESIAN_POINT('',(1.,-1.6,2.8));
#6620=CARTESIAN_POINT('',(3.,-1.6,2.8));
#6621=CARTESIAN_POINT('',(5.,-1.,2.8));
#6622=CARTESIAN_POINT('',(5.,-3.,2.8));
#6623=CARTESIAN_POINT('',(1.,-1.,2.8));
#6624=CARTESIAN_POINT('',(5.,-1.,2.8));
#6625=CARTESIAN_POINT('',(1.,-3.,2.8));
#6626=CARTESIAN_POINT('Origin',(3.,-1.,2.4));
#6627=CARTESIAN_POINT('',(5.,-1.,2.));
#6628=CARTESIAN_POINT('',(5.,-1.,2.));
#6629=CARTESIAN_POINT('',(1.,-1.,2.));
#6630=CARTESIAN_POINT('',(1.,-1.,2.));
#6631=CARTESIAN_POINT('',(1.,-1.,2.8));
#6632=CARTESIAN_POINT('Origin',(3.,-3.,2.4));
#6633=CARTESIAN_POINT('',(1.,-3.,2.));
#6634=CARTESIAN_POINT('',(1.,-3.,2.8));
#6635=CARTESIAN_POINT('',(5.,-3.,2.));
#6636=CARTESIAN_POINT('',(1.,-3.,2.));
#6637=CARTESIAN_POINT('',(5.,-3.,2.));
#6638=CARTESIAN_POINT('Origin',(5.,-1.6,2.));
#6639=CARTESIAN_POINT('',(5.,-1.6,2.));
#6640=CARTESIAN_POINT('',(1.,-1.6,2.));
#6641=CARTESIAN_POINT('Origin',(1.,-1.6,2.));
#6642=CARTESIAN_POINT('',(1.,-1.6,2.));
#6643=CARTESIAN_POINT('Origin',(5.,-2.4,2.));
#6644=CARTESIAN_POINT('',(5.,-3.,2.));
#6645=CARTESIAN_POINT('Origin',(3.,-2.,2.));
#7764=UNCERTAINTY_MEASURE_WITH_UNIT(LENGTH_MEASURE(0.001),#7807,
'DISTANCE_ACCURACY_VALUE',
'Maximum model space distance between geometric entities at asserted c
onnectivities');
#7782=UNCERTAINTY_MEASURE_WITH_UNIT(LENGTH_MEASURE(0.001),#7807,
'DISTANCE_ACCURACY_VALUE',
'Maximum model space distance between geometric entities at asserted c
onnectivities');
#7788=(
GEOMETRIC_REPRESENTATION_CONTEXT(3)
GLOBAL_UNCERTAINTY_ASSIGNED_CONTEXT((#7764))
GLOBAL_UNIT_ASSIGNED_CONTEXT((#7807,#7809,#7810))
REPRESENTATION_CONTEXT('','3D')
);
#7806=(
GEOMETRIC_REPRESENTATION_CONTEXT(3)
GLOBAL_UNCERTAINTY_ASSIGNED_CONTEXT((#7782))
GLOBAL_UNIT_ASSIGNED_CONTEXT((#7807,#7809,#7810))
REPRESENTATION_CONTEXT('','3D')
);
#7807=(
LENGTH_UNIT()
NAMED_UNIT(*)
SI_UNIT(.CENTI.,.METRE.)
);
#7809=(
NAMED_UNIT(*)
PLANE_ANGLE_UNIT()
SI_UNIT($,.RADIAN.)
);
#7810=(
NAMED_UNIT(*)
SI_UNIT($,.STERADIAN.)
SOLID_ANGLE_UNIT()
);
#7816=SHAPE_DEFINITION_REPRESENTATION(#7839,#7915);
#7839=PRODUCT_DEFINITION_SHAPE('',$,#7939);
#7915=SHAPE_REPRESENTATION('',(#4501),#7788);
#7933=PRODUCT_DEFINITION_CONTEXT('part definition',#8004,'design');
#7939=PRODUCT_DEFINITION('Axle Mount A','Axle Mount A',#7962,#7933);
#7962=PRODUCT_DEFINITION_FORMATION('',$,#8011);
#8004=APPLICATION_CONTEXT(
'Core Data for Automotive Mechanical Design Process');
#8005=PRODUCT_CONTEXT('part definition',#8004,'mechanical');
#8011=PRODUCT('Axle Mount A','Axle Mount A','Axle Mount A',(#8005));
#8085=COLOUR_RGB('Grey',0.48,0.52,0.57);
#8086=FILL_AREA_STYLE_COLOUR('',#8085);
#8087=FILL_AREA_STYLE('',(#8086));
#8088=SURFACE_STYLE_FILL_AREA(#8087);
#8089=SURFACE_SIDE_STYLE('',(#8088));
#8090=SURFACE_STYLE_USAGE(.BOTH.,#8089);
#8091=PRESENTATION_STYLE_ASSIGNMENT((#8090));
ENDSEC;
END-ISO-10303-21;
